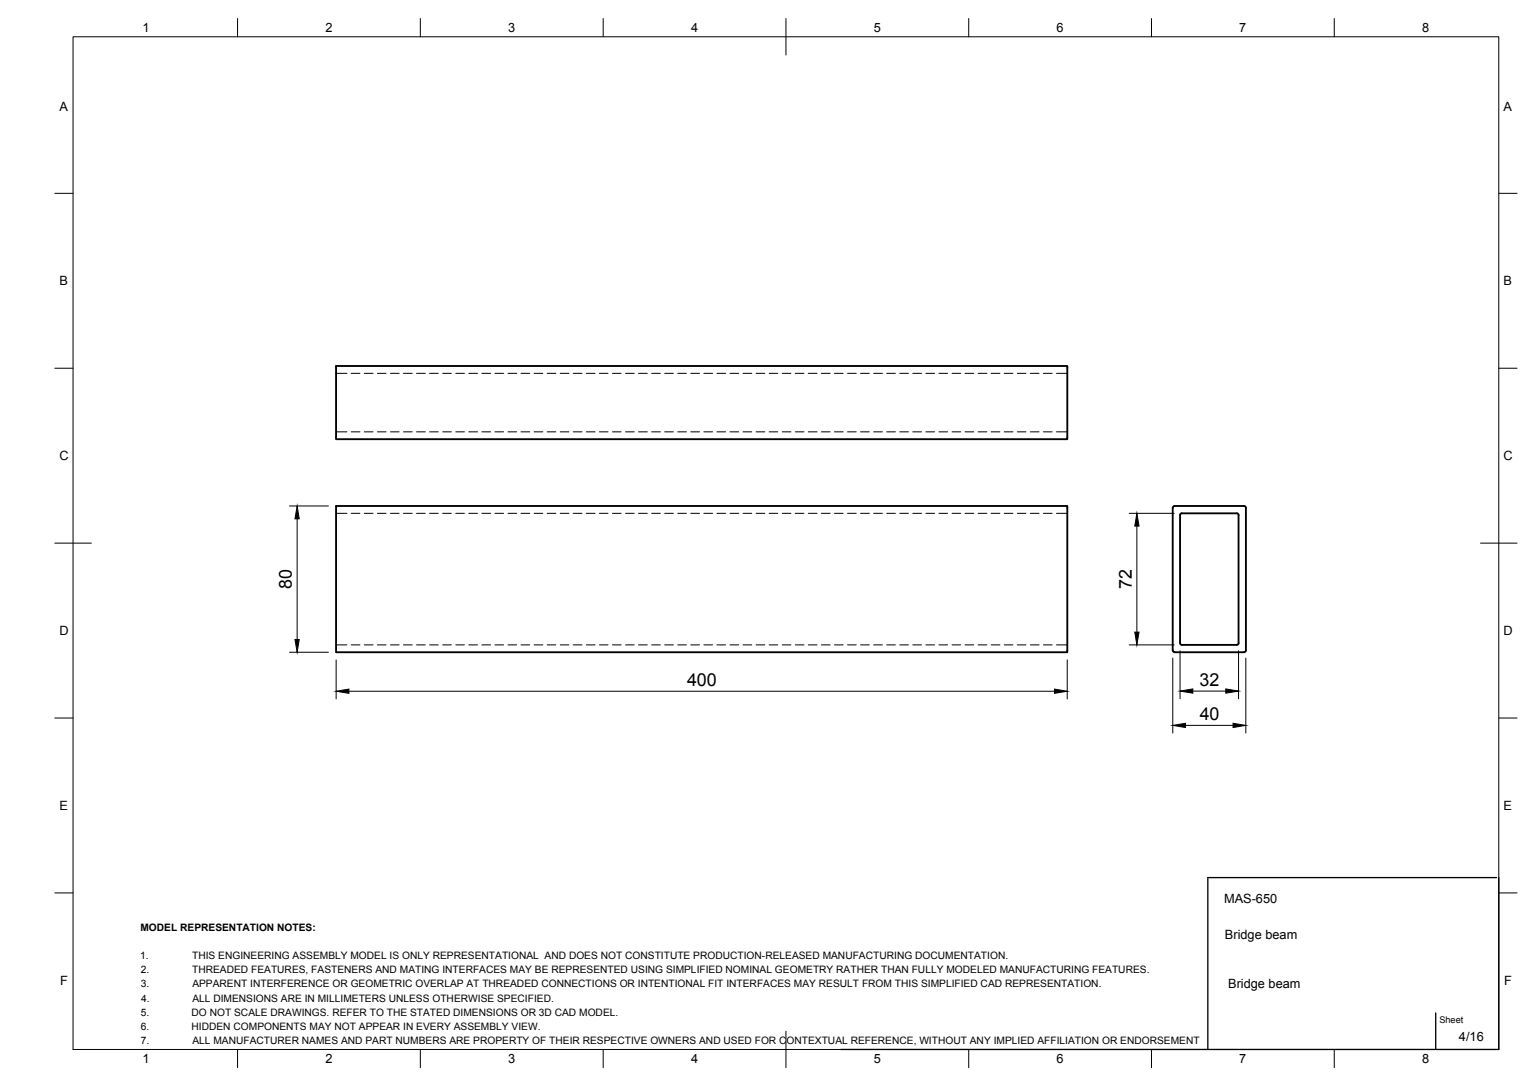
ISO-10303-21;
HEADER;
/* Generated by software containing ST-Developer
 * from STEP Tools, Inc. (www.steptools.com) 
 */

FILE_DESCRIPTION(
/* description */ ('Independent manual traversing gantry with native reusable aluminum pr
ofiles,180mm captured carriage travel, four bronze-bushed rollers, lin
ked ideal rolling motion, bonded acetal lateral guides, positive welde
d end stops and fully retained axle stacks. Editable native profile cu
t lengths220/400mm. Tool attachments viaM6 bridge-plate taps; mounted 
tool outside assembly. Welds, anchors, adhesives, fits, traction, load
/speed/structural/life ratings unassigned.'),
/* implementation_level */ '2;1');

FILE_NAME(
/* name */ 'Bridge beam.step',
/* time_stamp */ '2026-11-09T20:04:38-08:00',
/* author */ (''),
/* organization */ (''),
/* preprocessor_version */ 'ST-DEVELOPER v20.2',
/* originating_system */ 'Autodesk Translation Framework v15.17.0.0',
/* authorisation */ '');

FILE_SCHEMA (('AUTOMOTIVE_DESIGN { 1 0 10303 214 3 1 1 }'));
ENDSEC;

DATA;
#10=MECHANICAL_DESIGN_GEOMETRIC_PRESENTATION_REPRESENTATION('',(#471),#13231);
#439=SHAPE_REPRESENTATION_RELATIONSHIP('SRR','None',#13328,#455);
#455=ADVANCED_BREP_SHAPE_REPRESENTATION('',(#487),#13215);
#471=STYLED_ITEM('',(#13417),#487);
#487=MANIFOLD_SOLID_BREP('Aluminum rectangular hollow profile',#4151);
#503=FACE_BOUND('',#857,.T.);
#504=FACE_BOUND('',#873,.T.);
#552=PLANE('',#4349);
#553=PLANE('',#4350);
#554=PLANE('',#4360);
#555=PLANE('',#4367);
#556=PLANE('',#4370);
#557=PLANE('',#4373);
#558=PLANE('',#4376);
#559=PLANE('',#4377);
#560=PLANE('',#4378);
#561=PLANE('',#4379);
#633=FACE_OUTER_BOUND('',#854,.T.);
#634=FACE_OUTER_BOUND('',#855,.T.);
#635=FACE_OUTER_BOUND('',#856,.T.);
#636=FACE_OUTER_BOUND('',#858,.T.);
#637=FACE_OUTER_BOUND('',#859,.T.);
#638=FACE_OUTER_BOUND('',#860,.T.);
#639=FACE_OUTER_BOUND('',#861,.T.);
#640=FACE_OUTER_BOUND('',#862,.T.);
#641=FACE_OUTER_BOUND('',#863,.T.);
#642=FACE_OUTER_BOUND('',#864,.T.);
#643=FACE_OUTER_BOUND('',#865,.T.);
#644=FACE_OUTER_BOUND('',#866,.T.);
#645=FACE_OUTER_BOUND('',#867,.T.);
#646=FACE_OUTER_BOUND('',#868,.T.);
#647=FACE_OUTER_BOUND('',#869,.T.);
#648=FACE_OUTER_BOUND('',#870,.T.);
#649=FACE_OUTER_BOUND('',#871,.T.);
#650=FACE_OUTER_BOUND('',#872,.T.);
#854=EDGE_LOOP('',(#2682,#2683,#2684,#2685));
#855=EDGE_LOOP('',(#2686,#2687,#2688,#2689));
#856=EDGE_LOOP('',(#2690,#2691,#2692,#2693,#2694,#2695,#2696,#2697));
#857=EDGE_LOOP('',(#2698,#2699,#2700,#2701,#2702,#2703,#2704,#2705));
#858=EDGE_LOOP('',(#2706,#2707,#2708,#2709));
#859=EDGE_LOOP('',(#2710,#2711,#2712,#2713));
#860=EDGE_LOOP('',(#2714,#2715,#2716,#2717));
#861=EDGE_LOOP('',(#2718,#2719,#2720,#2721));
#862=EDGE_LOOP('',(#2722,#2723,#2724,#2725));
#863=EDGE_LOOP('',(#2726,#2727,#2728,#2729));
#864=EDGE_LOOP('',(#2730,#2731,#2732,#2733));
#865=EDGE_LOOP('',(#2734,#2735,#2736,#2737));
#866=EDGE_LOOP('',(#2738,#2739,#2740,#2741));
#867=EDGE_LOOP('',(#2742,#2743,#2744,#2745));
#868=EDGE_LOOP('',(#2746,#2747,#2748,#2749));
#869=EDGE_LOOP('',(#2750,#2751,#2752,#2753));
#870=EDGE_LOOP('',(#2754,#2755,#2756,#2757));
#871=EDGE_LOOP('',(#2758,#2759,#2760,#2761));
#872=EDGE_LOOP('',(#2762,#2763,#2764,#2765,#2766,#2767,#2768,#2769));
#873=EDGE_LOOP('',(#2770,#2771,#2772,#2773,#2774,#2775,#2776,#2777));
#1124=LINE('',#5786,#1386);
#1125=LINE('',#5789,#1387);
#1126=LINE('',#5792,#1388);
#1127=LINE('',#5794,#1389);
#1128=LINE('',#5795,#1390);
#1129=LINE('',#5798,#1391);
#1130=LINE('',#5802,#1392);
#1131=LINE('',#5806,#1393);
#1132=LINE('',#5810,#1394);
#1133=LINE('',#5814,#1395);
#1134=LINE('',#5818,#1396);
#1135=LINE('',#5822,#1397);
#1136=LINE('',#5826,#1398);
#1137=LINE('',#5829,#1399);
#1138=LINE('',#5832,#1400);
#1139=LINE('',#5833,#1401);
#1140=LINE('',#5837,#1402);
#1141=LINE('',#5840,#1403);
#1142=LINE('',#5846,#1404);
#1143=LINE('',#5847,#1405);
#1144=LINE('',#5850,#1406);
#1145=LINE('',#5851,#1407);
#1146=LINE('',#5855,#1408);
#1147=LINE('',#5858,#1409);
#1148=LINE('',#5859,#1410);
#1149=LINE('',#5863,#1411);
#1150=LINE('',#5866,#1412);
#1151=LINE('',#5867,#1413);
#1152=LINE('',#5871,#1414);
#1153=LINE('',#5873,#1415);
#1154=LINE('',#5875,#1416);
#1155=LINE('',#5877,#1417);
#1386=VECTOR('',#4743,10.);
#1387=VECTOR('',#4746,10.);
#1388=VECTOR('',#4749,10.);
#1389=VECTOR('',#4750,10.);
#1390=VECTOR('',#4751,10.);
#1391=VECTOR('',#4754,10.);
#1392=VECTOR('',#4757,10.);
#1393=VECTOR('',#4760,10.);
#1394=VECTOR('',#4763,10.);
#1395=VECTOR('',#4766,10.);
#1396=VECTOR('',#4769,10.);
#1397=VECTOR('',#4772,10.);
#1398=VECTOR('',#4777,10.);
#1399=VECTOR('',#4780,10.);
#1400=VECTOR('',#4783,10.);
#1401=VECTOR('',#4784,10.);
#1402=VECTOR('',#4789,10.);
#1403=VECTOR('',#4792,10.);
#1404=VECTOR('',#4799,10.);
#1405=VECTOR('',#4800,10.);
#1406=VECTOR('',#4803,10.);
#1407=VECTOR('',#4804,10.);
#1408=VECTOR('',#4809,10.);
#1409=VECTOR('',#4812,10.);
#1410=VECTOR('',#4813,10.);
#1411=VECTOR('',#4818,10.);
#1412=VECTOR('',#4821,10.);
#1413=VECTOR('',#4822,10.);
#1414=VECTOR('',#4827,10.);
#1415=VECTOR('',#4830,10.);
#1416=VECTOR('',#4833,10.);
#1417=VECTOR('',#4836,10.);
#1648=CIRCLE('',#4347,1.);
#1649=CIRCLE('',#4348,1.);
#1650=CIRCLE('',#4351,1.);
#1651=CIRCLE('',#4352,1.);
#1652=CIRCLE('',#4353,1.);
#1653=CIRCLE('',#4354,1.);
#1654=CIRCLE('',#4355,1.);
#1655=CIRCLE('',#4356,1.);
#1656=CIRCLE('',#4357,1.);
#1657=CIRCLE('',#4359,1.);
#1658=CIRCLE('',#4362,1.);
#1659=CIRCLE('',#4364,1.);
#1660=CIRCLE('',#4366,1.);
#1661=CIRCLE('',#4369,1.);
#1662=CIRCLE('',#4372,1.);
#1663=CIRCLE('',#4375,1.);
#1752=VERTEX_POINT('',#5782);
#1753=VERTEX_POINT('',#5783);
#1754=VERTEX_POINT('',#5785);
#1755=VERTEX_POINT('',#5787);
#1756=VERTEX_POINT('',#5791);
#1757=VERTEX_POINT('',#5793);
#1758=VERTEX_POINT('',#5797);
#1759=VERTEX_POINT('',#5799);
#1760=VERTEX_POINT('',#5801);
#1761=VERTEX_POINT('',#5803);
#1762=VERTEX_POINT('',#5805);
#1763=VERTEX_POINT('',#5808);
#1764=VERTEX_POINT('',#5809);
#1765=VERTEX_POINT('',#5811);
#1766=VERTEX_POINT('',#5813);
#1767=VERTEX_POINT('',#5815);
#1768=VERTEX_POINT('',#5817);
#1769=VERTEX_POINT('',#5819);
#1770=VERTEX_POINT('',#5821);
#1771=VERTEX_POINT('',#5825);
#1772=VERTEX_POINT('',#5827);
#1773=VERTEX_POINT('',#5831);
#1774=VERTEX_POINT('',#5835);
#1775=VERTEX_POINT('',#5839);
#1776=VERTEX_POINT('',#5843);
#1777=VERTEX_POINT('',#5844);
#1778=VERTEX_POINT('',#5849);
#1779=VERTEX_POINT('',#5853);
#1780=VERTEX_POINT('',#5857);
#1781=VERTEX_POINT('',#5861);
#1782=VERTEX_POINT('',#5865);
#1783=VERTEX_POINT('',#5869);
#2124=EDGE_CURVE('',#1752,#1753,#1648,.T.);
#2125=EDGE_CURVE('',#1753,#1754,#1124,.T.);
#2126=EDGE_CURVE('',#1754,#1755,#1649,.T.);
#2127=EDGE_CURVE('',#1755,#1752,#1125,.T.);
#2128=EDGE_CURVE('',#1756,#1753,#1126,.T.);
#2129=EDGE_CURVE('',#1757,#1756,#1127,.T.);
#2130=EDGE_CURVE('',#1757,#1754,#1128,.T.);
#2131=EDGE_CURVE('',#1752,#1758,#1129,.T.);
#2132=EDGE_CURVE('',#1759,#1758,#1650,.T.);
#2133=EDGE_CURVE('',#1759,#1760,#1130,.T.);
#2134=EDGE_CURVE('',#1761,#1760,#1651,.T.);
#2135=EDGE_CURVE('',#1761,#1762,#1131,.T.);
#2136=EDGE_CURVE('',#1756,#1762,#1652,.T.);
#2137=EDGE_CURVE('',#1763,#1764,#1132,.T.);
#2138=EDGE_CURVE('',#1765,#1764,#1653,.T.);
#2139=EDGE_CURVE('',#1765,#1766,#1133,.T.);
#2140=EDGE_CURVE('',#1767,#1766,#1654,.T.);
#2141=EDGE_CURVE('',#1767,#1768,#1134,.T.);
#2142=EDGE_CURVE('',#1769,#1768,#1655,.T.);
#2143=EDGE_CURVE('',#1769,#1770,#1135,.T.);
#2144=EDGE_CURVE('',#1763,#1770,#1656,.T.);
#2145=EDGE_CURVE('',#1758,#1771,#1136,.T.);
#2146=EDGE_CURVE('',#1771,#1772,#1657,.T.);
#2147=EDGE_CURVE('',#1772,#1759,#1137,.T.);
#2148=EDGE_CURVE('',#1772,#1773,#1138,.T.);
#2149=EDGE_CURVE('',#1760,#1773,#1139,.T.);
#2150=EDGE_CURVE('',#1773,#1774,#1658,.T.);
#2151=EDGE_CURVE('',#1774,#1761,#1140,.T.);
#2152=EDGE_CURVE('',#1762,#1775,#1141,.T.);
#2153=EDGE_CURVE('',#1775,#1757,#1659,.T.);
#2154=EDGE_CURVE('',#1776,#1777,#1660,.T.);
#2155=EDGE_CURVE('',#1777,#1765,#1142,.T.);
#2156=EDGE_CURVE('',#1764,#1776,#1143,.T.);
#2157=EDGE_CURVE('',#1777,#1778,#1144,.T.);
#2158=EDGE_CURVE('',#1766,#1778,#1145,.T.);
#2159=EDGE_CURVE('',#1778,#1779,#1661,.T.);
#2160=EDGE_CURVE('',#1779,#1767,#1146,.T.);
#2161=EDGE_CURVE('',#1779,#1780,#1147,.T.);
#2162=EDGE_CURVE('',#1768,#1780,#1148,.T.);
#2163=EDGE_CURVE('',#1780,#1781,#1662,.T.);
#2164=EDGE_CURVE('',#1781,#1769,#1149,.T.);
#2165=EDGE_CURVE('',#1781,#1782,#1150,.T.);
#2166=EDGE_CURVE('',#1770,#1782,#1151,.T.);
#2167=EDGE_CURVE('',#1782,#1783,#1663,.T.);
#2168=EDGE_CURVE('',#1783,#1763,#1152,.T.);
#2169=EDGE_CURVE('',#1783,#1776,#1153,.T.);
#2170=EDGE_CURVE('',#1774,#1775,#1154,.T.);
#2171=EDGE_CURVE('',#1755,#1771,#1155,.T.);
#2682=ORIENTED_EDGE('',*,*,#2124,.T.);
#2683=ORIENTED_EDGE('',*,*,#2125,.T.);
#2684=ORIENTED_EDGE('',*,*,#2126,.T.);
#2685=ORIENTED_EDGE('',*,*,#2127,.T.);
#2686=ORIENTED_EDGE('',*,*,#2125,.F.);
#2687=ORIENTED_EDGE('',*,*,#2128,.F.);
#2688=ORIENTED_EDGE('',*,*,#2129,.F.);
#2689=ORIENTED_EDGE('',*,*,#2130,.T.);
#2690=ORIENTED_EDGE('',*,*,#2124,.F.);
#2691=ORIENTED_EDGE('',*,*,#2131,.T.);
#2692=ORIENTED_EDGE('',*,*,#2132,.F.);
#2693=ORIENTED_EDGE('',*,*,#2133,.T.);
#2694=ORIENTED_EDGE('',*,*,#2134,.F.);
#2695=ORIENTED_EDGE('',*,*,#2135,.T.);
#2696=ORIENTED_EDGE('',*,*,#2136,.F.);
#2697=ORIENTED_EDGE('',*,*,#2128,.T.);
#2698=ORIENTED_EDGE('',*,*,#2137,.T.);
#2699=ORIENTED_EDGE('',*,*,#2138,.F.);
#2700=ORIENTED_EDGE('',*,*,#2139,.T.);
#2701=ORIENTED_EDGE('',*,*,#2140,.F.);
#2702=ORIENTED_EDGE('',*,*,#2141,.T.);
#2703=ORIENTED_EDGE('',*,*,#2142,.F.);
#2704=ORIENTED_EDGE('',*,*,#2143,.T.);
#2705=ORIENTED_EDGE('',*,*,#2144,.F.);
#2706=ORIENTED_EDGE('',*,*,#2132,.T.);
#2707=ORIENTED_EDGE('',*,*,#2145,.T.);
#2708=ORIENTED_EDGE('',*,*,#2146,.T.);
#2709=ORIENTED_EDGE('',*,*,#2147,.T.);
#2710=ORIENTED_EDGE('',*,*,#2147,.F.);
#2711=ORIENTED_EDGE('',*,*,#2148,.T.);
#2712=ORIENTED_EDGE('',*,*,#2149,.F.);
#2713=ORIENTED_EDGE('',*,*,#2133,.F.);
#2714=ORIENTED_EDGE('',*,*,#2134,.T.);
#2715=ORIENTED_EDGE('',*,*,#2149,.T.);
#2716=ORIENTED_EDGE('',*,*,#2150,.T.);
#2717=ORIENTED_EDGE('',*,*,#2151,.T.);
#2718=ORIENTED_EDGE('',*,*,#2136,.T.);
#2719=ORIENTED_EDGE('',*,*,#2152,.T.);
#2720=ORIENTED_EDGE('',*,*,#2153,.T.);
#2721=ORIENTED_EDGE('',*,*,#2129,.T.);
#2722=ORIENTED_EDGE('',*,*,#2154,.T.);
#2723=ORIENTED_EDGE('',*,*,#2155,.T.);
#2724=ORIENTED_EDGE('',*,*,#2138,.T.);
#2725=ORIENTED_EDGE('',*,*,#2156,.T.);
#2726=ORIENTED_EDGE('',*,*,#2155,.F.);
#2727=ORIENTED_EDGE('',*,*,#2157,.T.);
#2728=ORIENTED_EDGE('',*,*,#2158,.F.);
#2729=ORIENTED_EDGE('',*,*,#2139,.F.);
#2730=ORIENTED_EDGE('',*,*,#2159,.T.);
#2731=ORIENTED_EDGE('',*,*,#2160,.T.);
#2732=ORIENTED_EDGE('',*,*,#2140,.T.);
#2733=ORIENTED_EDGE('',*,*,#2158,.T.);
#2734=ORIENTED_EDGE('',*,*,#2160,.F.);
#2735=ORIENTED_EDGE('',*,*,#2161,.T.);
#2736=ORIENTED_EDGE('',*,*,#2162,.F.);
#2737=ORIENTED_EDGE('',*,*,#2141,.F.);
#2738=ORIENTED_EDGE('',*,*,#2163,.T.);
#2739=ORIENTED_EDGE('',*,*,#2164,.T.);
#2740=ORIENTED_EDGE('',*,*,#2142,.T.);
#2741=ORIENTED_EDGE('',*,*,#2162,.T.);
#2742=ORIENTED_EDGE('',*,*,#2164,.F.);
#2743=ORIENTED_EDGE('',*,*,#2165,.T.);
#2744=ORIENTED_EDGE('',*,*,#2166,.F.);
#2745=ORIENTED_EDGE('',*,*,#2143,.F.);
#2746=ORIENTED_EDGE('',*,*,#2167,.T.);
#2747=ORIENTED_EDGE('',*,*,#2168,.T.);
#2748=ORIENTED_EDGE('',*,*,#2144,.T.);
#2749=ORIENTED_EDGE('',*,*,#2166,.T.);
#2750=ORIENTED_EDGE('',*,*,#2156,.F.);
#2751=ORIENTED_EDGE('',*,*,#2137,.F.);
#2752=ORIENTED_EDGE('',*,*,#2168,.F.);
#2753=ORIENTED_EDGE('',*,*,#2169,.T.);
#2754=ORIENTED_EDGE('',*,*,#2151,.F.);
#2755=ORIENTED_EDGE('',*,*,#2170,.T.);
#2756=ORIENTED_EDGE('',*,*,#2152,.F.);
#2757=ORIENTED_EDGE('',*,*,#2135,.F.);
#2758=ORIENTED_EDGE('',*,*,#2127,.F.);
#2759=ORIENTED_EDGE('',*,*,#2171,.T.);
#2760=ORIENTED_EDGE('',*,*,#2145,.F.);
#2761=ORIENTED_EDGE('',*,*,#2131,.F.);
#2762=ORIENTED_EDGE('',*,*,#2126,.F.);
#2763=ORIENTED_EDGE('',*,*,#2130,.F.);
#2764=ORIENTED_EDGE('',*,*,#2153,.F.);
#2765=ORIENTED_EDGE('',*,*,#2170,.F.);
#2766=ORIENTED_EDGE('',*,*,#2150,.F.);
#2767=ORIENTED_EDGE('',*,*,#2148,.F.);
#2768=ORIENTED_EDGE('',*,*,#2146,.F.);
#2769=ORIENTED_EDGE('',*,*,#2171,.F.);
#2770=ORIENTED_EDGE('',*,*,#2167,.F.);
#2771=ORIENTED_EDGE('',*,*,#2165,.F.);
#2772=ORIENTED_EDGE('',*,*,#2163,.F.);
#2773=ORIENTED_EDGE('',*,*,#2161,.F.);
#2774=ORIENTED_EDGE('',*,*,#2159,.F.);
#2775=ORIENTED_EDGE('',*,*,#2157,.F.);
#2776=ORIENTED_EDGE('',*,*,#2154,.F.);
#2777=ORIENTED_EDGE('',*,*,#2169,.F.);
#3798=CYLINDRICAL_SURFACE('',#4346,1.);
#3799=CYLINDRICAL_SURFACE('',#4358,1.);
#3800=CYLINDRICAL_SURFACE('',#4361,1.);
#3801=CYLINDRICAL_SURFACE('',#4363,1.);
#3802=CYLINDRICAL_SURFACE('',#4365,1.);
#3803=CYLINDRICAL_SURFACE('',#4368,1.);
#3804=CYLINDRICAL_SURFACE('',#4371,1.);
#3805=CYLINDRICAL_SURFACE('',#4374,1.);
#3930=ADVANCED_FACE('',(#633),#3798,.T.);
#3931=ADVANCED_FACE('',(#634),#552,.T.);
#3932=ADVANCED_FACE('',(#635,#503),#553,.T.);
#3933=ADVANCED_FACE('',(#636),#3799,.T.);
#3934=ADVANCED_FACE('',(#637),#554,.T.);
#3935=ADVANCED_FACE('',(#638),#3800,.T.);
#3936=ADVANCED_FACE('',(#639),#3801,.T.);
#3937=ADVANCED_FACE('',(#640),#3802,.F.);
#3938=ADVANCED_FACE('',(#641),#555,.T.);
#3939=ADVANCED_FACE('',(#642),#3803,.F.);
#3940=ADVANCED_FACE('',(#643),#556,.T.);
#3941=ADVANCED_FACE('',(#644),#3804,.F.);
#3942=ADVANCED_FACE('',(#645),#557,.T.);
#3943=ADVANCED_FACE('',(#646),#3805,.F.);
#3944=ADVANCED_FACE('',(#647),#558,.T.);
#3945=ADVANCED_FACE('',(#648),#559,.T.);
#3946=ADVANCED_FACE('',(#649),#560,.T.);
#3947=ADVANCED_FACE('',(#650,#504),#561,.F.);
#4151=CLOSED_SHELL('',(#3930,#3931,#3932,#3933,#3934,#3935,#3936,#3937,
#3938,#3939,#3940,#3941,#3942,#3943,#3944,#3945,#3946,#3947));
#4345=AXIS2_PLACEMENT_3D('',#5780,#4737,#4738);
#4346=AXIS2_PLACEMENT_3D('',#5781,#4739,#4740);
#4347=AXIS2_PLACEMENT_3D('',#5784,#4741,#4742);
#4348=AXIS2_PLACEMENT_3D('',#5788,#4744,#4745);
#4349=AXIS2_PLACEMENT_3D('',#5790,#4747,#4748);
#4350=AXIS2_PLACEMENT_3D('',#5796,#4752,#4753);
#4351=AXIS2_PLACEMENT_3D('',#5800,#4755,#4756);
#4352=AXIS2_PLACEMENT_3D('',#5804,#4758,#4759);
#4353=AXIS2_PLACEMENT_3D('',#5807,#4761,#4762);
#4354=AXIS2_PLACEMENT_3D('',#5812,#4764,#4765);
#4355=AXIS2_PLACEMENT_3D('',#5816,#4767,#4768);
#4356=AXIS2_PLACEMENT_3D('',#5820,#4770,#4771);
#4357=AXIS2_PLACEMENT_3D('',#5823,#4773,#4774);
#4358=AXIS2_PLACEMENT_3D('',#5824,#4775,#4776);
#4359=AXIS2_PLACEMENT_3D('',#5828,#4778,#4779);
#4360=AXIS2_PLACEMENT_3D('',#5830,#4781,#4782);
#4361=AXIS2_PLACEMENT_3D('',#5834,#4785,#4786);
#4362=AXIS2_PLACEMENT_3D('',#5836,#4787,#4788);
#4363=AXIS2_PLACEMENT_3D('',#5838,#4790,#4791);
#4364=AXIS2_PLACEMENT_3D('',#5841,#4793,#4794);
#4365=AXIS2_PLACEMENT_3D('',#5842,#4795,#4796);
#4366=AXIS2_PLACEMENT_3D('',#5845,#4797,#4798);
#4367=AXIS2_PLACEMENT_3D('',#5848,#4801,#4802);
#4368=AXIS2_PLACEMENT_3D('',#5852,#4805,#4806);
#4369=AXIS2_PLACEMENT_3D('',#5854,#4807,#4808);
#4370=AXIS2_PLACEMENT_3D('',#5856,#4810,#4811);
#4371=AXIS2_PLACEMENT_3D('',#5860,#4814,#4815);
#4372=AXIS2_PLACEMENT_3D('',#5862,#4816,#4817);
#4373=AXIS2_PLACEMENT_3D('',#5864,#4819,#4820);
#4374=AXIS2_PLACEMENT_3D('',#5868,#4823,#4824);
#4375=AXIS2_PLACEMENT_3D('',#5870,#4825,#4826);
#4376=AXIS2_PLACEMENT_3D('',#5872,#4828,#4829);
#4377=AXIS2_PLACEMENT_3D('',#5874,#4831,#4832);
#4378=AXIS2_PLACEMENT_3D('',#5876,#4834,#4835);
#4379=AXIS2_PLACEMENT_3D('',#5878,#4837,#4838);
#4737=DIRECTION('axis',(0.,0.,1.));
#4738=DIRECTION('refdir',(1.,0.,0.));
#4739=DIRECTION('center_axis',(0.,0.,1.));
#4740=DIRECTION('ref_axis',(-0.707106781186546,-0.707106781186549,0.));
#4741=DIRECTION('center_axis',(0.,0.,-1.));
#4742=DIRECTION('ref_axis',(-0.707106781186546,-0.707106781186549,0.));
#4743=DIRECTION('',(0.,0.,-1.));
#4744=DIRECTION('center_axis',(0.,0.,1.));
#4745=DIRECTION('ref_axis',(-0.707106781186546,-0.707106781186549,0.));
#4746=DIRECTION('',(0.,0.,1.));
#4747=DIRECTION('center_axis',(-1.,0.,0.));
#4748=DIRECTION('ref_axis',(0.,-1.,0.));
#4749=DIRECTION('',(0.,-1.,0.));
#4750=DIRECTION('',(0.,0.,1.));
#4751=DIRECTION('',(0.,-1.,0.));
#4752=DIRECTION('center_axis',(0.,0.,1.));
#4753=DIRECTION('ref_axis',(1.,0.,0.));
#4754=DIRECTION('',(1.,0.,0.));
#4755=DIRECTION('center_axis',(0.,0.,-1.));
#4756=DIRECTION('ref_axis',(0.707106781186546,-0.707106781186549,0.));
#4757=DIRECTION('',(0.,1.,0.));
#4758=DIRECTION('center_axis',(0.,0.,-1.));
#4759=DIRECTION('ref_axis',(0.707106781186546,0.707106781186549,0.));
#4760=DIRECTION('',(-1.,0.,0.));
#4761=DIRECTION('center_axis',(0.,0.,-1.));
#4762=DIRECTION('ref_axis',(-0.707106781186546,0.707106781186549,0.));
#4763=DIRECTION('',(0.,1.,0.));
#4764=DIRECTION('center_axis',(0.,0.,1.));
#4765=DIRECTION('ref_axis',(-0.707106781186546,0.707106781186549,0.));
#4766=DIRECTION('',(1.,0.,0.));
#4767=DIRECTION('center_axis',(0.,0.,1.));
#4768=DIRECTION('ref_axis',(0.707106781186546,0.707106781186549,0.));
#4769=DIRECTION('',(0.,-1.,0.));
#4770=DIRECTION('center_axis',(0.,0.,1.));
#4771=DIRECTION('ref_axis',(0.707106781186546,-0.707106781186549,0.));
#4772=DIRECTION('',(-1.,0.,0.));
#4773=DIRECTION('center_axis',(0.,0.,1.));
#4774=DIRECTION('ref_axis',(-0.707106781186546,-0.707106781186549,0.));
#4775=DIRECTION('center_axis',(0.,0.,1.));
#4776=DIRECTION('ref_axis',(0.707106781186546,-0.707106781186549,0.));
#4777=DIRECTION('',(0.,0.,-1.));
#4778=DIRECTION('center_axis',(0.,0.,1.));
#4779=DIRECTION('ref_axis',(0.707106781186546,-0.707106781186549,0.));
#4780=DIRECTION('',(0.,0.,1.));
#4781=DIRECTION('center_axis',(1.,0.,0.));
#4782=DIRECTION('ref_axis',(0.,1.,0.));
#4783=DIRECTION('',(0.,1.,0.));
#4784=DIRECTION('',(0.,0.,-1.));
#4785=DIRECTION('center_axis',(0.,0.,1.));
#4786=DIRECTION('ref_axis',(0.707106781186546,0.707106781186549,0.));
#4787=DIRECTION('center_axis',(0.,0.,1.));
#4788=DIRECTION('ref_axis',(0.707106781186546,0.707106781186549,0.));
#4789=DIRECTION('',(0.,0.,1.));
#4790=DIRECTION('center_axis',(0.,0.,1.));
#4791=DIRECTION('ref_axis',(-0.707106781186546,0.707106781186549,0.));
#4792=DIRECTION('',(0.,0.,-1.));
#4793=DIRECTION('center_axis',(0.,0.,1.));
#4794=DIRECTION('ref_axis',(-0.707106781186546,0.707106781186549,0.));
#4795=DIRECTION('center_axis',(0.,0.,1.));
#4796=DIRECTION('ref_axis',(-0.707106781186546,0.707106781186549,0.));
#4797=DIRECTION('center_axis',(0.,0.,-1.));
#4798=DIRECTION('ref_axis',(-0.707106781186546,0.707106781186549,0.));
#4799=DIRECTION('',(0.,0.,1.));
#4800=DIRECTION('',(0.,0.,-1.));
#4801=DIRECTION('center_axis',(0.,-1.,0.));
#4802=DIRECTION('ref_axis',(1.,0.,0.));
#4803=DIRECTION('',(1.,0.,0.));
#4804=DIRECTION('',(0.,0.,-1.));
#4805=DIRECTION('center_axis',(0.,0.,1.));
#4806=DIRECTION('ref_axis',(0.707106781186546,0.707106781186549,0.));
#4807=DIRECTION('center_axis',(0.,0.,-1.));
#4808=DIRECTION('ref_axis',(0.707106781186546,0.707106781186549,0.));
#4809=DIRECTION('',(0.,0.,1.));
#4810=DIRECTION('center_axis',(-1.,0.,0.));
#4811=DIRECTION('ref_axis',(0.,-1.,0.));
#4812=DIRECTION('',(0.,-1.,0.));
#4813=DIRECTION('',(0.,0.,-1.));
#4814=DIRECTION('center_axis',(0.,0.,1.));
#4815=DIRECTION('ref_axis',(0.707106781186546,-0.707106781186549,0.));
#4816=DIRECTION('center_axis',(0.,0.,-1.));
#4817=DIRECTION('ref_axis',(0.707106781186546,-0.707106781186549,0.));
#4818=DIRECTION('',(0.,0.,1.));
#4819=DIRECTION('center_axis',(0.,1.,0.));
#4820=DIRECTION('ref_axis',(-1.,0.,0.));
#4821=DIRECTION('',(-1.,0.,0.));
#4822=DIRECTION('',(0.,0.,-1.));
#4823=DIRECTION('center_axis',(0.,0.,1.));
#4824=DIRECTION('ref_axis',(-0.707106781186546,-0.707106781186549,0.));
#4825=DIRECTION('center_axis',(0.,0.,-1.));
#4826=DIRECTION('ref_axis',(-0.707106781186546,-0.707106781186549,0.));
#4827=DIRECTION('',(0.,0.,1.));
#4828=DIRECTION('center_axis',(1.,0.,0.));
#4829=DIRECTION('ref_axis',(0.,1.,0.));
#4830=DIRECTION('',(0.,1.,0.));
#4831=DIRECTION('center_axis',(0.,1.,0.));
#4832=DIRECTION('ref_axis',(-1.,0.,0.));
#4833=DIRECTION('',(-1.,0.,0.));
#4834=DIRECTION('center_axis',(0.,-1.,0.));
#4835=DIRECTION('ref_axis',(1.,0.,0.));
#4836=DIRECTION('',(1.,0.,0.));
#4837=DIRECTION('center_axis',(0.,0.,1.));
#4838=DIRECTION('ref_axis',(1.,0.,0.));
#5780=CARTESIAN_POINT('',(0.,0.,0.));
#5781=CARTESIAN_POINT('Origin',(-39.,-19.,0.));
#5782=CARTESIAN_POINT('',(-39.,-20.,400.));
#5783=CARTESIAN_POINT('',(-40.,-19.,400.));
#5784=CARTESIAN_POINT('Origin',(-39.,-19.,400.));
#5785=CARTESIAN_POINT('',(-40.,-19.,0.));
#5786=CARTESIAN_POINT('',(-40.,-19.,0.));
#5787=CARTESIAN_POINT('',(-39.,-20.,0.));
#5788=CARTESIAN_POINT('Origin',(-39.,-19.,0.));
#5789=CARTESIAN_POINT('',(-39.,-20.,0.));
#5790=CARTESIAN_POINT('Origin',(-40.,20.,0.));
#5791=CARTESIAN_POINT('',(-40.,19.,400.));
#5792=CARTESIAN_POINT('',(-40.,20.,400.));
#5793=CARTESIAN_POINT('',(-40.,19.,0.));
#5794=CARTESIAN_POINT('',(-40.,19.,0.));
#5795=CARTESIAN_POINT('',(-40.,20.,0.));
#5796=CARTESIAN_POINT('Origin',(0.,0.,400.));
#5797=CARTESIAN_POINT('',(39.,-20.,400.));
#5798=CARTESIAN_POINT('',(-40.,-20.,400.));
#5799=CARTESIAN_POINT('',(40.,-19.,400.));
#5800=CARTESIAN_POINT('Origin',(39.,-19.,400.));
#5801=CARTESIAN_POINT('',(40.,19.,400.));
#5802=CARTESIAN_POINT('',(40.,-20.,400.));
#5803=CARTESIAN_POINT('',(39.,20.,400.));
#5804=CARTESIAN_POINT('Origin',(39.,19.,400.));
#5805=CARTESIAN_POINT('',(-39.,20.,400.));
#5806=CARTESIAN_POINT('',(40.,20.,400.));
#5807=CARTESIAN_POINT('Origin',(-39.,19.,400.));
#5808=CARTESIAN_POINT('',(-36.,-15.,400.));
#5809=CARTESIAN_POINT('',(-36.,15.,400.));
#5810=CARTESIAN_POINT('',(-36.,16.,400.));
#5811=CARTESIAN_POINT('',(-35.,16.,400.));
#5812=CARTESIAN_POINT('Origin',(-35.,15.,400.));
#5813=CARTESIAN_POINT('',(35.,16.,400.));
#5814=CARTESIAN_POINT('',(36.,16.,400.));
#5815=CARTESIAN_POINT('',(36.,15.,400.));
#5816=CARTESIAN_POINT('Origin',(35.,15.,400.));
#5817=CARTESIAN_POINT('',(36.,-15.,400.));
#5818=CARTESIAN_POINT('',(36.,-16.,400.));
#5819=CARTESIAN_POINT('',(35.,-16.,400.));
#5820=CARTESIAN_POINT('Origin',(35.,-15.,400.));
#5821=CARTESIAN_POINT('',(-35.,-16.,400.));
#5822=CARTESIAN_POINT('',(-36.,-16.,400.));
#5823=CARTESIAN_POINT('Origin',(-35.,-15.,400.));
#5824=CARTESIAN_POINT('Origin',(39.,-19.,0.));
#5825=CARTESIAN_POINT('',(39.,-20.,0.));
#5826=CARTESIAN_POINT('',(39.,-20.,0.));
#5827=CARTESIAN_POINT('',(40.,-19.,0.));
#5828=CARTESIAN_POINT('Origin',(39.,-19.,0.));
#5829=CARTESIAN_POINT('',(40.,-19.,0.));
#5830=CARTESIAN_POINT('Origin',(40.,-20.,0.));
#5831=CARTESIAN_POINT('',(40.,19.,0.));
#5832=CARTESIAN_POINT('',(40.,-20.,0.));
#5833=CARTESIAN_POINT('',(40.,19.,0.));
#5834=CARTESIAN_POINT('Origin',(39.,19.,0.));
#5835=CARTESIAN_POINT('',(39.,20.,0.));
#5836=CARTESIAN_POINT('Origin',(39.,19.,0.));
#5837=CARTESIAN_POINT('',(39.,20.,0.));
#5838=CARTESIAN_POINT('Origin',(-39.,19.,0.));
#5839=CARTESIAN_POINT('',(-39.,20.,0.));
#5840=CARTESIAN_POINT('',(-39.,20.,0.));
#5841=CARTESIAN_POINT('Origin',(-39.,19.,0.));
#5842=CARTESIAN_POINT('Origin',(-35.,15.,0.));
#5843=CARTESIAN_POINT('',(-36.,15.,0.));
#5844=CARTESIAN_POINT('',(-35.,16.,0.));
#5845=CARTESIAN_POINT('Origin',(-35.,15.,0.));
#5846=CARTESIAN_POINT('',(-35.,16.,0.));
#5847=CARTESIAN_POINT('',(-36.,15.,0.));
#5848=CARTESIAN_POINT('Origin',(-36.,16.,0.));
#5849=CARTESIAN_POINT('',(35.,16.,0.));
#5850=CARTESIAN_POINT('',(36.,16.,0.));
#5851=CARTESIAN_POINT('',(35.,16.,0.));
#5852=CARTESIAN_POINT('Origin',(35.,15.,0.));
#5853=CARTESIAN_POINT('',(36.,15.,0.));
#5854=CARTESIAN_POINT('Origin',(35.,15.,0.));
#5855=CARTESIAN_POINT('',(36.,15.,0.));
#5856=CARTESIAN_POINT('Origin',(36.,16.,0.));
#5857=CARTESIAN_POINT('',(36.,-15.,0.));
#5858=CARTESIAN_POINT('',(36.,-16.,0.));
#5859=CARTESIAN_POINT('',(36.,-15.,0.));
#5860=CARTESIAN_POINT('Origin',(35.,-15.,0.));
#5861=CARTESIAN_POINT('',(35.,-16.,0.));
#5862=CARTESIAN_POINT('Origin',(35.,-15.,0.));
#5863=CARTESIAN_POINT('',(35.,-16.,0.));
#5864=CARTESIAN_POINT('Origin',(36.,-16.,0.));
#5865=CARTESIAN_POINT('',(-35.,-16.,0.));
#5866=CARTESIAN_POINT('',(-36.,-16.,0.));
#5867=CARTESIAN_POINT('',(-35.,-16.,0.));
#5868=CARTESIAN_POINT('Origin',(-35.,-15.,0.));
#5869=CARTESIAN_POINT('',(-36.,-15.,0.));
#5870=CARTESIAN_POINT('Origin',(-35.,-15.,0.));
#5871=CARTESIAN_POINT('',(-36.,-15.,0.));
#5872=CARTESIAN_POINT('Origin',(-36.,-16.,0.));
#5873=CARTESIAN_POINT('',(-36.,16.,0.));
#5874=CARTESIAN_POINT('Origin',(40.,20.,0.));
#5875=CARTESIAN_POINT('',(40.,20.,0.));
#5876=CARTESIAN_POINT('Origin',(-40.,-20.,0.));
#5877=CARTESIAN_POINT('',(-40.,-20.,0.));
#5878=CARTESIAN_POINT('Origin',(0.,0.,0.));
#13197=UNCERTAINTY_MEASURE_WITH_UNIT(LENGTH_MEASURE(0.01),#13232,
'DISTANCE_ACCURACY_VALUE',
'Maximum model space distance between geometric entities at asserted c
onnectivities');
#13213=UNCERTAINTY_MEASURE_WITH_UNIT(LENGTH_MEASURE(0.01),#13232,
'DISTANCE_ACCURACY_VALUE',
'Maximum model space distance between geometric entities at asserted c
onnectivities');
#13215=(
GEOMETRIC_REPRESENTATION_CONTEXT(3)
GLOBAL_UNCERTAINTY_ASSIGNED_CONTEXT((#13197))
GLOBAL_UNIT_ASSIGNED_CONTEXT((#13232,#13234,#13235))
REPRESENTATION_CONTEXT('','3D')
);
#13231=(
GEOMETRIC_REPRESENTATION_CONTEXT(3)
GLOBAL_UNCERTAINTY_ASSIGNED_CONTEXT((#13213))
GLOBAL_UNIT_ASSIGNED_CONTEXT((#13232,#13234,#13235))
REPRESENTATION_CONTEXT('','3D')
);
#13232=(
LENGTH_UNIT()
NAMED_UNIT(*)
SI_UNIT(.MILLI.,.METRE.)
);
#13234=(
NAMED_UNIT(*)
PLANE_ANGLE_UNIT()
SI_UNIT($,.RADIAN.)
);
#13235=(
NAMED_UNIT(*)
SI_UNIT($,.STERADIAN.)
SOLID_ANGLE_UNIT()
);
#13237=SHAPE_DEFINITION_REPRESENTATION(#13254,#13328);
#13254=PRODUCT_DEFINITION_SHAPE('',$,#13346);
#13328=SHAPE_REPRESENTATION('',(#4345),#13215);
#13344=PRODUCT_DEFINITION_CONTEXT('part definition',#13397,'design');
#13346=PRODUCT_DEFINITION('Bridge beam','Bridge beam',#13363,#13344);
#13363=PRODUCT_DEFINITION_FORMATION('',$,#13400);
#13397=APPLICATION_CONTEXT(
'Core Data for Automotive Mechanical Design Process');
#13398=PRODUCT_CONTEXT('part definition',#13397,'mechanical');
#13400=PRODUCT('Bridge beam','Bridge beam',
'Independent aluminum extrusion section. Whole-mm nominal die dimensio
ns; parametric saw-cut length. Select structural loading, tolerances a
nd finish for the assembly application.',(#13398));
#13417=PRESENTATION_STYLE_ASSIGNMENT((#13431));
#13431=SURFACE_STYLE_USAGE(.BOTH.,#13445);
#13445=SURFACE_SIDE_STYLE('',(#13459));
#13459=SURFACE_STYLE_FILL_AREA(#13473);
#13473=FILL_AREA_STYLE('Dark blue',(#13487));
#13487=FILL_AREA_STYLE_COLOUR('Dark blue',#13501);
#13501=COLOUR_RGB('Dark blue',0.0901960784313725,0.270588235294118,0.513725490196078);
ENDSEC;
END-ISO-10303-21;
